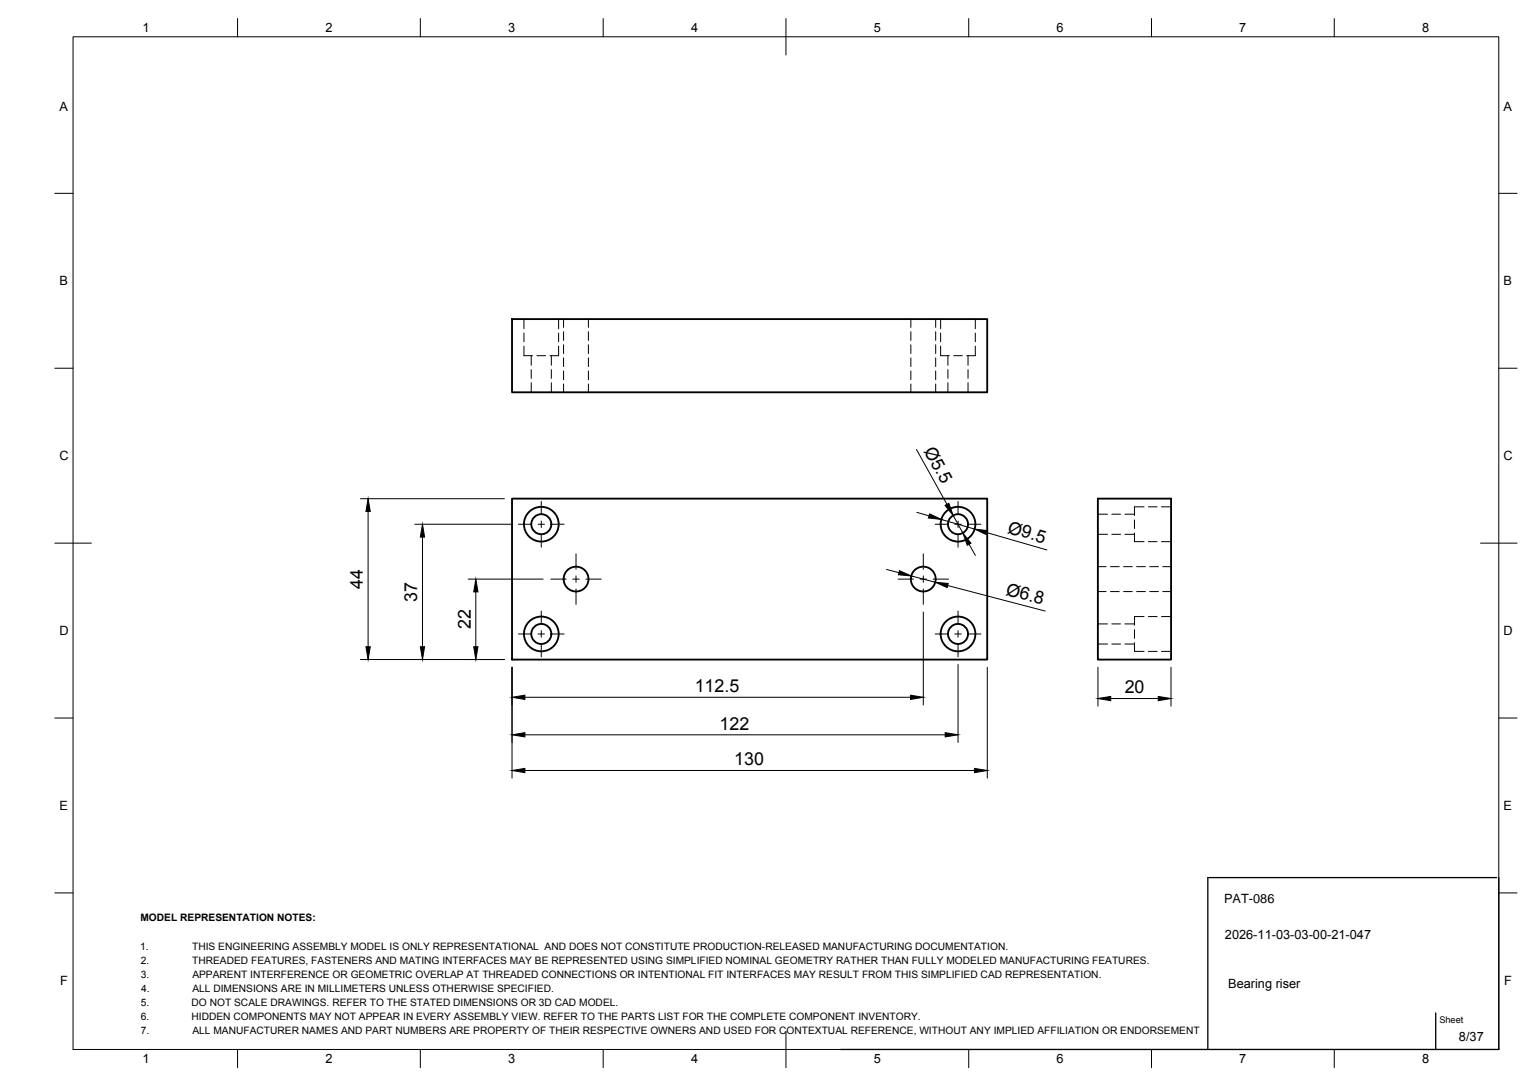
ISO-10303-21;
HEADER;
/* Generated by software containing ST-Developer
 * from STEP Tools, Inc. (www.steptools.com) 
 */

FILE_DESCRIPTION(
/* description */ ('Ratchet and pawl hand winch drum'),
/* implementation_level */ '2;1');

FILE_NAME(
/* name */ 'Bearing riser.step',
/* time_stamp */ '2026-10-27T12:42:58-07:00',
/* author */ (''),
/* organization */ (''),
/* preprocessor_version */ 'ST-DEVELOPER v20.2',
/* originating_system */ 'Autodesk Translation Framework v15.17.0.0',
/* authorisation */ '');

FILE_SCHEMA (('AUTOMOTIVE_DESIGN { 1 0 10303 214 3 1 1 }'));
ENDSEC;

DATA;
#10=MECHANICAL_DESIGN_GEOMETRIC_PRESENTATION_REPRESENTATION('',(#392),#11801);
#324=SHAPE_REPRESENTATION_RELATIONSHIP('SRR','None',#11950,#358);
#358=ADVANCED_BREP_SHAPE_REPRESENTATION('',(#427),#11767);
#392=STYLED_ITEM('',(#12213),#427);
#427=MANIFOLD_SOLID_BREP('Body1',#6269);
#476=FACE_BOUND('',#1246,.T.);
#477=FACE_BOUND('',#1249,.T.);
#478=FACE_BOUND('',#1254,.T.);
#479=FACE_BOUND('',#1257,.T.);
#480=FACE_BOUND('',#1267,.T.);
#481=FACE_BOUND('',#1268,.T.);
#482=FACE_BOUND('',#1269,.T.);
#483=FACE_BOUND('',#1270,.T.);
#484=FACE_BOUND('',#1271,.T.);
#485=FACE_BOUND('',#1272,.T.);
#486=FACE_BOUND('',#1274,.T.);
#487=FACE_BOUND('',#1275,.T.);
#488=FACE_BOUND('',#1276,.T.);
#489=FACE_BOUND('',#1277,.T.);
#490=FACE_BOUND('',#1278,.T.);
#491=FACE_BOUND('',#1279,.T.);
#619=PLANE('',#6736);
#620=PLANE('',#6741);
#621=PLANE('',#6750);
#622=PLANE('',#6755);
#623=PLANE('',#6767);
#624=PLANE('',#6768);
#625=PLANE('',#6769);
#626=PLANE('',#6770);
#627=PLANE('',#6771);
#628=PLANE('',#6772);
#868=FACE_OUTER_BOUND('',#1244,.T.);
#869=FACE_OUTER_BOUND('',#1245,.T.);
#870=FACE_OUTER_BOUND('',#1247,.T.);
#871=FACE_OUTER_BOUND('',#1248,.T.);
#872=FACE_OUTER_BOUND('',#1250,.T.);
#873=FACE_OUTER_BOUND('',#1251,.T.);
#874=FACE_OUTER_BOUND('',#1252,.T.);
#875=FACE_OUTER_BOUND('',#1253,.T.);
#876=FACE_OUTER_BOUND('',#1255,.T.);
#877=FACE_OUTER_BOUND('',#1256,.T.);
#878=FACE_OUTER_BOUND('',#1258,.T.);
#879=FACE_OUTER_BOUND('',#1259,.T.);
#880=FACE_OUTER_BOUND('',#1260,.T.);
#881=FACE_OUTER_BOUND('',#1261,.T.);
#882=FACE_OUTER_BOUND('',#1262,.T.);
#883=FACE_OUTER_BOUND('',#1263,.T.);
#884=FACE_OUTER_BOUND('',#1264,.T.);
#885=FACE_OUTER_BOUND('',#1265,.T.);
#886=FACE_OUTER_BOUND('',#1266,.T.);
#887=FACE_OUTER_BOUND('',#1273,.T.);
#1244=EDGE_LOOP('',(#4379,#4380,#4381,#4382));
#1245=EDGE_LOOP('',(#4383));
#1246=EDGE_LOOP('',(#4384));
#1247=EDGE_LOOP('',(#4385,#4386,#4387,#4388));
#1248=EDGE_LOOP('',(#4389));
#1249=EDGE_LOOP('',(#4390));
#1250=EDGE_LOOP('',(#4391,#4392,#4393,#4394));
#1251=EDGE_LOOP('',(#4395,#4396,#4397,#4398));
#1252=EDGE_LOOP('',(#4399,#4400,#4401,#4402));
#1253=EDGE_LOOP('',(#4403));
#1254=EDGE_LOOP('',(#4404));
#1255=EDGE_LOOP('',(#4405,#4406,#4407,#4408));
#1256=EDGE_LOOP('',(#4409));
#1257=EDGE_LOOP('',(#4410));
#1258=EDGE_LOOP('',(#4411,#4412,#4413,#4414));
#1259=EDGE_LOOP('',(#4415,#4416,#4417,#4418));
#1260=EDGE_LOOP('',(#4419,#4420,#4421,#4422));
#1261=EDGE_LOOP('',(#4423,#4424,#4425,#4426));
#1262=EDGE_LOOP('',(#4427,#4428,#4429,#4430));
#1263=EDGE_LOOP('',(#4431,#4432,#4433,#4434));
#1264=EDGE_LOOP('',(#4435,#4436,#4437,#4438));
#1265=EDGE_LOOP('',(#4439,#4440,#4441,#4442));
#1266=EDGE_LOOP('',(#4443,#4444,#4445,#4446));
#1267=EDGE_LOOP('',(#4447));
#1268=EDGE_LOOP('',(#4448));
#1269=EDGE_LOOP('',(#4449));
#1270=EDGE_LOOP('',(#4450));
#1271=EDGE_LOOP('',(#4451));
#1272=EDGE_LOOP('',(#4452));
#1273=EDGE_LOOP('',(#4453,#4454,#4455,#4456));
#1274=EDGE_LOOP('',(#4457));
#1275=EDGE_LOOP('',(#4458));
#1276=EDGE_LOOP('',(#4459));
#1277=EDGE_LOOP('',(#4460));
#1278=EDGE_LOOP('',(#4461));
#1279=EDGE_LOOP('',(#4462));
#1743=LINE('',#9375,#2254);
#1744=LINE('',#9384,#2255);
#1745=LINE('',#9392,#2256);
#1746=LINE('',#9396,#2257);
#1747=LINE('',#9401,#2258);
#1748=LINE('',#9410,#2259);
#1749=LINE('',#9418,#2260);
#1750=LINE('',#9422,#2261);
#1751=LINE('',#9427,#2262);
#1752=LINE('',#9433,#2263);
#1753=LINE('',#9438,#2264);
#1754=LINE('',#9440,#2265);
#1755=LINE('',#9442,#2266);
#1756=LINE('',#9443,#2267);
#1757=LINE('',#9446,#2268);
#1758=LINE('',#9448,#2269);
#1759=LINE('',#9449,#2270);
#1760=LINE('',#9452,#2271);
#1761=LINE('',#9454,#2272);
#1762=LINE('',#9455,#2273);
#1763=LINE('',#9457,#2274);
#1764=LINE('',#9458,#2275);
#2254=VECTOR('',#7516,0.475);
#2255=VECTOR('',#7527,0.475);
#2256=VECTOR('',#7538,0.275);
#2257=VECTOR('',#7543,0.275);
#2258=VECTOR('',#7548,0.475);
#2259=VECTOR('',#7559,0.475);
#2260=VECTOR('',#7570,0.275);
#2261=VECTOR('',#7575,0.275);
#2262=VECTOR('',#7580,0.34);
#2263=VECTOR('',#7587,0.34);
#2264=VECTOR('',#7592,1.);
#2265=VECTOR('',#7593,1.);
#2266=VECTOR('',#7594,1.);
#2267=VECTOR('',#7595,1.);
#2268=VECTOR('',#7598,1.);
#2269=VECTOR('',#7599,1.);
#2270=VECTOR('',#7600,1.);
#2271=VECTOR('',#7603,1.);
#2272=VECTOR('',#7604,1.);
#2273=VECTOR('',#7605,1.);
#2274=VECTOR('',#7608,1.);
#2275=VECTOR('',#7609,1.);
#2739=CIRCLE('',#6734,0.475);
#2740=CIRCLE('',#6735,0.475);
#2741=CIRCLE('',#6737,0.275);
#2742=CIRCLE('',#6739,0.475);
#2743=CIRCLE('',#6740,0.475);
#2744=CIRCLE('',#6742,0.275);
#2745=CIRCLE('',#6744,0.275);
#2746=CIRCLE('',#6746,0.275);
#2747=CIRCLE('',#6748,0.475);
#2748=CIRCLE('',#6749,0.475);
#2749=CIRCLE('',#6751,0.275);
#2750=CIRCLE('',#6753,0.475);
#2751=CIRCLE('',#6754,0.475);
#2752=CIRCLE('',#6756,0.275);
#2753=CIRCLE('',#6758,0.275);
#2754=CIRCLE('',#6760,0.275);
#2755=CIRCLE('',#6762,0.34);
#2756=CIRCLE('',#6763,0.34);
#2757=CIRCLE('',#6765,0.34);
#2758=CIRCLE('',#6766,0.34);
#2986=VERTEX_POINT('',#9372);
#2987=VERTEX_POINT('',#9374);
#2988=VERTEX_POINT('',#9378);
#2989=VERTEX_POINT('',#9381);
#2990=VERTEX_POINT('',#9383);
#2991=VERTEX_POINT('',#9387);
#2992=VERTEX_POINT('',#9390);
#2993=VERTEX_POINT('',#9394);
#2994=VERTEX_POINT('',#9398);
#2995=VERTEX_POINT('',#9400);
#2996=VERTEX_POINT('',#9404);
#2997=VERTEX_POINT('',#9407);
#2998=VERTEX_POINT('',#9409);
#2999=VERTEX_POINT('',#9413);
#3000=VERTEX_POINT('',#9416);
#3001=VERTEX_POINT('',#9420);
#3002=VERTEX_POINT('',#9424);
#3003=VERTEX_POINT('',#9426);
#3004=VERTEX_POINT('',#9430);
#3005=VERTEX_POINT('',#9432);
#3006=VERTEX_POINT('',#9436);
#3007=VERTEX_POINT('',#9437);
#3008=VERTEX_POINT('',#9439);
#3009=VERTEX_POINT('',#9441);
#3010=VERTEX_POINT('',#9445);
#3011=VERTEX_POINT('',#9447);
#3012=VERTEX_POINT('',#9451);
#3013=VERTEX_POINT('',#9453);
#3533=EDGE_CURVE('',#2986,#2986,#2739,.T.);
#3534=EDGE_CURVE('',#2986,#2987,#1743,.T.);
#3535=EDGE_CURVE('',#2987,#2987,#2740,.T.);
#3536=EDGE_CURVE('',#2988,#2988,#2741,.T.);
#3537=EDGE_CURVE('',#2989,#2989,#2742,.T.);
#3538=EDGE_CURVE('',#2989,#2990,#1744,.T.);
#3539=EDGE_CURVE('',#2990,#2990,#2743,.T.);
#3540=EDGE_CURVE('',#2991,#2991,#2744,.T.);
#3541=EDGE_CURVE('',#2992,#2992,#2745,.T.);
#3542=EDGE_CURVE('',#2992,#2988,#1745,.T.);
#3543=EDGE_CURVE('',#2993,#2993,#2746,.T.);
#3544=EDGE_CURVE('',#2993,#2991,#1746,.T.);
#3545=EDGE_CURVE('',#2994,#2994,#2747,.T.);
#3546=EDGE_CURVE('',#2994,#2995,#1747,.T.);
#3547=EDGE_CURVE('',#2995,#2995,#2748,.T.);
#3548=EDGE_CURVE('',#2996,#2996,#2749,.T.);
#3549=EDGE_CURVE('',#2997,#2997,#2750,.T.);
#3550=EDGE_CURVE('',#2997,#2998,#1748,.T.);
#3551=EDGE_CURVE('',#2998,#2998,#2751,.T.);
#3552=EDGE_CURVE('',#2999,#2999,#2752,.T.);
#3553=EDGE_CURVE('',#3000,#3000,#2753,.T.);
#3554=EDGE_CURVE('',#3000,#2996,#1749,.T.);
#3555=EDGE_CURVE('',#3001,#3001,#2754,.T.);
#3556=EDGE_CURVE('',#3001,#2999,#1750,.T.);
#3557=EDGE_CURVE('',#3002,#3002,#2755,.T.);
#3558=EDGE_CURVE('',#3002,#3003,#1751,.T.);
#3559=EDGE_CURVE('',#3003,#3003,#2756,.T.);
#3560=EDGE_CURVE('',#3004,#3004,#2757,.T.);
#3561=EDGE_CURVE('',#3004,#3005,#1752,.T.);
#3562=EDGE_CURVE('',#3005,#3005,#2758,.T.);
#3563=EDGE_CURVE('',#3006,#3007,#1753,.T.);
#3564=EDGE_CURVE('',#3007,#3008,#1754,.T.);
#3565=EDGE_CURVE('',#3009,#3008,#1755,.T.);
#3566=EDGE_CURVE('',#3006,#3009,#1756,.T.);
#3567=EDGE_CURVE('',#3010,#3006,#1757,.T.);
#3568=EDGE_CURVE('',#3011,#3009,#1758,.T.);
#3569=EDGE_CURVE('',#3010,#3011,#1759,.T.);
#3570=EDGE_CURVE('',#3012,#3010,#1760,.T.);
#3571=EDGE_CURVE('',#3013,#3011,#1761,.T.);
#3572=EDGE_CURVE('',#3012,#3013,#1762,.T.);
#3573=EDGE_CURVE('',#3007,#3012,#1763,.T.);
#3574=EDGE_CURVE('',#3008,#3013,#1764,.T.);
#4379=ORIENTED_EDGE('',*,*,#3533,.F.);
#4380=ORIENTED_EDGE('',*,*,#3534,.T.);
#4381=ORIENTED_EDGE('',*,*,#3535,.F.);
#4382=ORIENTED_EDGE('',*,*,#3534,.F.);
#4383=ORIENTED_EDGE('',*,*,#3533,.T.);
#4384=ORIENTED_EDGE('',*,*,#3536,.F.);
#4385=ORIENTED_EDGE('',*,*,#3537,.F.);
#4386=ORIENTED_EDGE('',*,*,#3538,.T.);
#4387=ORIENTED_EDGE('',*,*,#3539,.F.);
#4388=ORIENTED_EDGE('',*,*,#3538,.F.);
#4389=ORIENTED_EDGE('',*,*,#3537,.T.);
#4390=ORIENTED_EDGE('',*,*,#3540,.F.);
#4391=ORIENTED_EDGE('',*,*,#3541,.F.);
#4392=ORIENTED_EDGE('',*,*,#3542,.T.);
#4393=ORIENTED_EDGE('',*,*,#3536,.T.);
#4394=ORIENTED_EDGE('',*,*,#3542,.F.);
#4395=ORIENTED_EDGE('',*,*,#3543,.F.);
#4396=ORIENTED_EDGE('',*,*,#3544,.T.);
#4397=ORIENTED_EDGE('',*,*,#3540,.T.);
#4398=ORIENTED_EDGE('',*,*,#3544,.F.);
#4399=ORIENTED_EDGE('',*,*,#3545,.F.);
#4400=ORIENTED_EDGE('',*,*,#3546,.T.);
#4401=ORIENTED_EDGE('',*,*,#3547,.F.);
#4402=ORIENTED_EDGE('',*,*,#3546,.F.);
#4403=ORIENTED_EDGE('',*,*,#3545,.T.);
#4404=ORIENTED_EDGE('',*,*,#3548,.F.);
#4405=ORIENTED_EDGE('',*,*,#3549,.F.);
#4406=ORIENTED_EDGE('',*,*,#3550,.T.);
#4407=ORIENTED_EDGE('',*,*,#3551,.F.);
#4408=ORIENTED_EDGE('',*,*,#3550,.F.);
#4409=ORIENTED_EDGE('',*,*,#3549,.T.);
#4410=ORIENTED_EDGE('',*,*,#3552,.F.);
#4411=ORIENTED_EDGE('',*,*,#3553,.F.);
#4412=ORIENTED_EDGE('',*,*,#3554,.T.);
#4413=ORIENTED_EDGE('',*,*,#3548,.T.);
#4414=ORIENTED_EDGE('',*,*,#3554,.F.);
#4415=ORIENTED_EDGE('',*,*,#3555,.F.);
#4416=ORIENTED_EDGE('',*,*,#3556,.T.);
#4417=ORIENTED_EDGE('',*,*,#3552,.T.);
#4418=ORIENTED_EDGE('',*,*,#3556,.F.);
#4419=ORIENTED_EDGE('',*,*,#3557,.F.);
#4420=ORIENTED_EDGE('',*,*,#3558,.T.);
#4421=ORIENTED_EDGE('',*,*,#3559,.F.);
#4422=ORIENTED_EDGE('',*,*,#3558,.F.);
#4423=ORIENTED_EDGE('',*,*,#3560,.F.);
#4424=ORIENTED_EDGE('',*,*,#3561,.T.);
#4425=ORIENTED_EDGE('',*,*,#3562,.F.);
#4426=ORIENTED_EDGE('',*,*,#3561,.F.);
#4427=ORIENTED_EDGE('',*,*,#3563,.T.);
#4428=ORIENTED_EDGE('',*,*,#3564,.T.);
#4429=ORIENTED_EDGE('',*,*,#3565,.F.);
#4430=ORIENTED_EDGE('',*,*,#3566,.F.);
#4431=ORIENTED_EDGE('',*,*,#3567,.T.);
#4432=ORIENTED_EDGE('',*,*,#3566,.T.);
#4433=ORIENTED_EDGE('',*,*,#3568,.F.);
#4434=ORIENTED_EDGE('',*,*,#3569,.F.);
#4435=ORIENTED_EDGE('',*,*,#3570,.T.);
#4436=ORIENTED_EDGE('',*,*,#3569,.T.);
#4437=ORIENTED_EDGE('',*,*,#3571,.F.);
#4438=ORIENTED_EDGE('',*,*,#3572,.F.);
#4439=ORIENTED_EDGE('',*,*,#3573,.T.);
#4440=ORIENTED_EDGE('',*,*,#3572,.T.);
#4441=ORIENTED_EDGE('',*,*,#3574,.F.);
#4442=ORIENTED_EDGE('',*,*,#3564,.F.);
#4443=ORIENTED_EDGE('',*,*,#3574,.T.);
#4444=ORIENTED_EDGE('',*,*,#3571,.T.);
#4445=ORIENTED_EDGE('',*,*,#3568,.T.);
#4446=ORIENTED_EDGE('',*,*,#3565,.T.);
#4447=ORIENTED_EDGE('',*,*,#3562,.T.);
#4448=ORIENTED_EDGE('',*,*,#3559,.T.);
#4449=ORIENTED_EDGE('',*,*,#3551,.T.);
#4450=ORIENTED_EDGE('',*,*,#3547,.T.);
#4451=ORIENTED_EDGE('',*,*,#3539,.T.);
#4452=ORIENTED_EDGE('',*,*,#3535,.T.);
#4453=ORIENTED_EDGE('',*,*,#3573,.F.);
#4454=ORIENTED_EDGE('',*,*,#3563,.F.);
#4455=ORIENTED_EDGE('',*,*,#3567,.F.);
#4456=ORIENTED_EDGE('',*,*,#3570,.F.);
#4457=ORIENTED_EDGE('',*,*,#3541,.T.);
#4458=ORIENTED_EDGE('',*,*,#3543,.T.);
#4459=ORIENTED_EDGE('',*,*,#3553,.T.);
#4460=ORIENTED_EDGE('',*,*,#3555,.T.);
#4461=ORIENTED_EDGE('',*,*,#3557,.T.);
#4462=ORIENTED_EDGE('',*,*,#3560,.T.);
#5817=CYLINDRICAL_SURFACE('',#6733,0.475);
#5818=CYLINDRICAL_SURFACE('',#6738,0.475);
#5819=CYLINDRICAL_SURFACE('',#6743,0.275);
#5820=CYLINDRICAL_SURFACE('',#6745,0.275);
#5821=CYLINDRICAL_SURFACE('',#6747,0.475);
#5822=CYLINDRICAL_SURFACE('',#6752,0.475);
#5823=CYLINDRICAL_SURFACE('',#6757,0.275);
#5824=CYLINDRICAL_SURFACE('',#6759,0.275);
#5825=CYLINDRICAL_SURFACE('',#6761,0.34);
#5826=CYLINDRICAL_SURFACE('',#6764,0.34);
#5938=ADVANCED_FACE('',(#868),#5817,.F.);
#5939=ADVANCED_FACE('',(#869,#476),#619,.T.);
#5940=ADVANCED_FACE('',(#870),#5818,.F.);
#5941=ADVANCED_FACE('',(#871,#477),#620,.T.);
#5942=ADVANCED_FACE('',(#872),#5819,.F.);
#5943=ADVANCED_FACE('',(#873),#5820,.F.);
#5944=ADVANCED_FACE('',(#874),#5821,.F.);
#5945=ADVANCED_FACE('',(#875,#478),#621,.T.);
#5946=ADVANCED_FACE('',(#876),#5822,.F.);
#5947=ADVANCED_FACE('',(#877,#479),#622,.T.);
#5948=ADVANCED_FACE('',(#878),#5823,.F.);
#5949=ADVANCED_FACE('',(#879),#5824,.F.);
#5950=ADVANCED_FACE('',(#880),#5825,.F.);
#5951=ADVANCED_FACE('',(#881),#5826,.F.);
#5952=ADVANCED_FACE('',(#882),#623,.T.);
#5953=ADVANCED_FACE('',(#883),#624,.T.);
#5954=ADVANCED_FACE('',(#884),#625,.T.);
#5955=ADVANCED_FACE('',(#885),#626,.T.);
#5956=ADVANCED_FACE('',(#886,#480,#481,#482,#483,#484,#485),#627,.T.);
#5957=ADVANCED_FACE('',(#887,#486,#487,#488,#489,#490,#491),#628,.F.);
#6269=CLOSED_SHELL('',(#5938,#5939,#5940,#5941,#5942,#5943,#5944,#5945,
#5946,#5947,#5948,#5949,#5950,#5951,#5952,#5953,#5954,#5955,#5956,#5957));
#6732=AXIS2_PLACEMENT_3D('',#9370,#7510,#7511);
#6733=AXIS2_PLACEMENT_3D('',#9371,#7512,#7513);
#6734=AXIS2_PLACEMENT_3D('',#9373,#7514,#7515);
#6735=AXIS2_PLACEMENT_3D('',#9376,#7517,#7518);
#6736=AXIS2_PLACEMENT_3D('',#9377,#7519,#7520);
#6737=AXIS2_PLACEMENT_3D('',#9379,#7521,#7522);
#6738=AXIS2_PLACEMENT_3D('',#9380,#7523,#7524);
#6739=AXIS2_PLACEMENT_3D('',#9382,#7525,#7526);
#6740=AXIS2_PLACEMENT_3D('',#9385,#7528,#7529);
#6741=AXIS2_PLACEMENT_3D('',#9386,#7530,#7531);
#6742=AXIS2_PLACEMENT_3D('',#9388,#7532,#7533);
#6743=AXIS2_PLACEMENT_3D('',#9389,#7534,#7535);
#6744=AXIS2_PLACEMENT_3D('',#9391,#7536,#7537);
#6745=AXIS2_PLACEMENT_3D('',#9393,#7539,#7540);
#6746=AXIS2_PLACEMENT_3D('',#9395,#7541,#7542);
#6747=AXIS2_PLACEMENT_3D('',#9397,#7544,#7545);
#6748=AXIS2_PLACEMENT_3D('',#9399,#7546,#7547);
#6749=AXIS2_PLACEMENT_3D('',#9402,#7549,#7550);
#6750=AXIS2_PLACEMENT_3D('',#9403,#7551,#7552);
#6751=AXIS2_PLACEMENT_3D('',#9405,#7553,#7554);
#6752=AXIS2_PLACEMENT_3D('',#9406,#7555,#7556);
#6753=AXIS2_PLACEMENT_3D('',#9408,#7557,#7558);
#6754=AXIS2_PLACEMENT_3D('',#9411,#7560,#7561);
#6755=AXIS2_PLACEMENT_3D('',#9412,#7562,#7563);
#6756=AXIS2_PLACEMENT_3D('',#9414,#7564,#7565);
#6757=AXIS2_PLACEMENT_3D('',#9415,#7566,#7567);
#6758=AXIS2_PLACEMENT_3D('',#9417,#7568,#7569);
#6759=AXIS2_PLACEMENT_3D('',#9419,#7571,#7572);
#6760=AXIS2_PLACEMENT_3D('',#9421,#7573,#7574);
#6761=AXIS2_PLACEMENT_3D('',#9423,#7576,#7577);
#6762=AXIS2_PLACEMENT_3D('',#9425,#7578,#7579);
#6763=AXIS2_PLACEMENT_3D('',#9428,#7581,#7582);
#6764=AXIS2_PLACEMENT_3D('',#9429,#7583,#7584);
#6765=AXIS2_PLACEMENT_3D('',#9431,#7585,#7586);
#6766=AXIS2_PLACEMENT_3D('',#9434,#7588,#7589);
#6767=AXIS2_PLACEMENT_3D('',#9435,#7590,#7591);
#6768=AXIS2_PLACEMENT_3D('',#9444,#7596,#7597);
#6769=AXIS2_PLACEMENT_3D('',#9450,#7601,#7602);
#6770=AXIS2_PLACEMENT_3D('',#9456,#7606,#7607);
#6771=AXIS2_PLACEMENT_3D('',#9459,#7610,#7611);
#6772=AXIS2_PLACEMENT_3D('',#9460,#7612,#7613);
#7510=DIRECTION('axis',(0.,0.,1.));
#7511=DIRECTION('refdir',(1.,0.,0.));
#7512=DIRECTION('center_axis',(0.,0.,1.));
#7513=DIRECTION('ref_axis',(1.,0.,0.));
#7514=DIRECTION('center_axis',(0.,0.,1.));
#7515=DIRECTION('ref_axis',(1.,0.,0.));
#7516=DIRECTION('',(0.,0.,1.));
#7517=DIRECTION('center_axis',(0.,0.,-1.));
#7518=DIRECTION('ref_axis',(1.,0.,0.));
#7519=DIRECTION('center_axis',(0.,0.,1.));
#7520=DIRECTION('ref_axis',(1.,0.,0.));
#7521=DIRECTION('center_axis',(0.,0.,1.));
#7522=DIRECTION('ref_axis',(1.,0.,0.));
#7523=DIRECTION('center_axis',(0.,0.,1.));
#7524=DIRECTION('ref_axis',(1.,0.,0.));
#7525=DIRECTION('center_axis',(0.,0.,1.));
#7526=DIRECTION('ref_axis',(1.,0.,0.));
#7527=DIRECTION('',(0.,0.,1.));
#7528=DIRECTION('center_axis',(0.,0.,-1.));
#7529=DIRECTION('ref_axis',(1.,0.,0.));
#7530=DIRECTION('center_axis',(0.,0.,1.));
#7531=DIRECTION('ref_axis',(1.,0.,0.));
#7532=DIRECTION('center_axis',(0.,0.,1.));
#7533=DIRECTION('ref_axis',(1.,0.,0.));
#7534=DIRECTION('center_axis',(0.,0.,1.));
#7535=DIRECTION('ref_axis',(1.,0.,0.));
#7536=DIRECTION('center_axis',(0.,0.,1.));
#7537=DIRECTION('ref_axis',(1.,0.,0.));
#7538=DIRECTION('',(0.,0.,1.));
#7539=DIRECTION('center_axis',(0.,0.,1.));
#7540=DIRECTION('ref_axis',(1.,0.,0.));
#7541=DIRECTION('center_axis',(0.,0.,1.));
#7542=DIRECTION('ref_axis',(1.,0.,0.));
#7543=DIRECTION('',(0.,0.,1.));
#7544=DIRECTION('center_axis',(0.,0.,1.));
#7545=DIRECTION('ref_axis',(1.,0.,0.));
#7546=DIRECTION('center_axis',(0.,0.,1.));
#7547=DIRECTION('ref_axis',(1.,0.,0.));
#7548=DIRECTION('',(0.,0.,1.));
#7549=DIRECTION('center_axis',(0.,0.,-1.));
#7550=DIRECTION('ref_axis',(1.,0.,0.));
#7551=DIRECTION('center_axis',(0.,0.,1.));
#7552=DIRECTION('ref_axis',(1.,0.,0.));
#7553=DIRECTION('center_axis',(0.,0.,1.));
#7554=DIRECTION('ref_axis',(1.,0.,0.));
#7555=DIRECTION('center_axis',(0.,0.,1.));
#7556=DIRECTION('ref_axis',(1.,0.,0.));
#7557=DIRECTION('center_axis',(0.,0.,1.));
#7558=DIRECTION('ref_axis',(1.,0.,0.));
#7559=DIRECTION('',(0.,0.,1.));
#7560=DIRECTION('center_axis',(0.,0.,-1.));
#7561=DIRECTION('ref_axis',(1.,0.,0.));
#7562=DIRECTION('center_axis',(0.,0.,1.));
#7563=DIRECTION('ref_axis',(1.,0.,0.));
#7564=DIRECTION('center_axis',(0.,0.,1.));
#7565=DIRECTION('ref_axis',(1.,0.,0.));
#7566=DIRECTION('center_axis',(0.,0.,1.));
#7567=DIRECTION('ref_axis',(1.,0.,0.));
#7568=DIRECTION('center_axis',(0.,0.,1.));
#7569=DIRECTION('ref_axis',(1.,0.,0.));
#7570=DIRECTION('',(0.,0.,1.));
#7571=DIRECTION('center_axis',(0.,0.,1.));
#7572=DIRECTION('ref_axis',(1.,0.,0.));
#7573=DIRECTION('center_axis',(0.,0.,1.));
#7574=DIRECTION('ref_axis',(1.,0.,0.));
#7575=DIRECTION('',(0.,0.,1.));
#7576=DIRECTION('center_axis',(0.,0.,1.));
#7577=DIRECTION('ref_axis',(1.,0.,0.));
#7578=DIRECTION('center_axis',(0.,0.,1.));
#7579=DIRECTION('ref_axis',(1.,0.,0.));
#7580=DIRECTION('',(0.,0.,1.));
#7581=DIRECTION('center_axis',(0.,0.,-1.));
#7582=DIRECTION('ref_axis',(1.,0.,0.));
#7583=DIRECTION('center_axis',(0.,0.,1.));
#7584=DIRECTION('ref_axis',(1.,0.,0.));
#7585=DIRECTION('center_axis',(0.,0.,1.));
#7586=DIRECTION('ref_axis',(1.,0.,0.));
#7587=DIRECTION('',(0.,0.,1.));
#7588=DIRECTION('center_axis',(0.,0.,-1.));
#7589=DIRECTION('ref_axis',(1.,0.,0.));
#7590=DIRECTION('center_axis',(0.,1.,0.));
#7591=DIRECTION('ref_axis',(-1.,0.,0.));
#7592=DIRECTION('',(-1.,0.,0.));
#7593=DIRECTION('',(0.,0.,1.));
#7594=DIRECTION('',(-1.,0.,0.));
#7595=DIRECTION('',(0.,0.,1.));
#7596=DIRECTION('center_axis',(1.,0.,0.));
#7597=DIRECTION('ref_axis',(0.,1.,0.));
#7598=DIRECTION('',(0.,1.,0.));
#7599=DIRECTION('',(0.,1.,0.));
#7600=DIRECTION('',(0.,0.,1.));
#7601=DIRECTION('center_axis',(0.,-1.,0.));
#7602=DIRECTION('ref_axis',(1.,0.,0.));
#7603=DIRECTION('',(1.,0.,0.));
#7604=DIRECTION('',(1.,0.,0.));
#7605=DIRECTION('',(0.,0.,1.));
#7606=DIRECTION('center_axis',(-1.,0.,0.));
#7607=DIRECTION('ref_axis',(0.,-1.,0.));
#7608=DIRECTION('',(0.,-1.,0.));
#7609=DIRECTION('',(0.,-1.,0.));
#7610=DIRECTION('center_axis',(0.,0.,1.));
#7611=DIRECTION('ref_axis',(1.,0.,0.));
#7612=DIRECTION('center_axis',(0.,0.,1.));
#7613=DIRECTION('ref_axis',(1.,0.,0.));
#9370=CARTESIAN_POINT('',(0.,0.,0.));
#9371=CARTESIAN_POINT('Origin',(5.7,-1.5,2.2));
#9372=CARTESIAN_POINT('',(5.225,-1.5,2.2));
#9373=CARTESIAN_POINT('Origin',(5.7,-1.5,2.2));
#9374=CARTESIAN_POINT('',(5.225,-1.5,3.2));
#9375=CARTESIAN_POINT('',(5.225,-1.5,2.2));
#9376=CARTESIAN_POINT('Origin',(5.7,-1.5,3.2));
#9377=CARTESIAN_POINT('Origin',(5.7,-1.5,2.2));
#9378=CARTESIAN_POINT('',(5.425,-1.5,2.2));
#9379=CARTESIAN_POINT('Origin',(5.7,-1.5,2.2));
#9380=CARTESIAN_POINT('Origin',(5.7,1.5,2.2));
#9381=CARTESIAN_POINT('',(5.225,1.5,2.2));
#9382=CARTESIAN_POINT('Origin',(5.7,1.5,2.2));
#9383=CARTESIAN_POINT('',(5.225,1.5,3.2));
#9384=CARTESIAN_POINT('',(5.225,1.5,2.2));
#9385=CARTESIAN_POINT('Origin',(5.7,1.5,3.2));
#9386=CARTESIAN_POINT('Origin',(5.7,1.5,2.2));
#9387=CARTESIAN_POINT('',(5.425,1.5,2.2));
#9388=CARTESIAN_POINT('Origin',(5.7,1.5,2.2));
#9389=CARTESIAN_POINT('Origin',(5.7,-1.5,1.1));
#9390=CARTESIAN_POINT('',(5.425,-1.5,1.2));
#9391=CARTESIAN_POINT('Origin',(5.7,-1.5,1.2));
#9392=CARTESIAN_POINT('',(5.425,-1.5,1.1));
#9393=CARTESIAN_POINT('Origin',(5.7,1.5,1.1));
#9394=CARTESIAN_POINT('',(5.425,1.5,1.2));
#9395=CARTESIAN_POINT('Origin',(5.7,1.5,1.2));
#9396=CARTESIAN_POINT('',(5.425,1.5,1.1));
#9397=CARTESIAN_POINT('Origin',(-5.7,-1.5,2.2));
#9398=CARTESIAN_POINT('',(-6.175,-1.5,2.2));
#9399=CARTESIAN_POINT('Origin',(-5.7,-1.5,2.2));
#9400=CARTESIAN_POINT('',(-6.175,-1.5,3.2));
#9401=CARTESIAN_POINT('',(-6.175,-1.5,2.2));
#9402=CARTESIAN_POINT('Origin',(-5.7,-1.5,3.2));
#9403=CARTESIAN_POINT('Origin',(-5.7,-1.5,2.2));
#9404=CARTESIAN_POINT('',(-5.975,-1.5,2.2));
#9405=CARTESIAN_POINT('Origin',(-5.7,-1.5,2.2));
#9406=CARTESIAN_POINT('Origin',(-5.7,1.5,2.2));
#9407=CARTESIAN_POINT('',(-6.175,1.5,2.2));
#9408=CARTESIAN_POINT('Origin',(-5.7,1.5,2.2));
#9409=CARTESIAN_POINT('',(-6.175,1.5,3.2));
#9410=CARTESIAN_POINT('',(-6.175,1.5,2.2));
#9411=CARTESIAN_POINT('Origin',(-5.7,1.5,3.2));
#9412=CARTESIAN_POINT('Origin',(-5.7,1.5,2.2));
#9413=CARTESIAN_POINT('',(-5.975,1.5,2.2));
#9414=CARTESIAN_POINT('Origin',(-5.7,1.5,2.2));
#9415=CARTESIAN_POINT('Origin',(-5.7,-1.5,1.1));
#9416=CARTESIAN_POINT('',(-5.975,-1.5,1.2));
#9417=CARTESIAN_POINT('Origin',(-5.7,-1.5,1.2));
#9418=CARTESIAN_POINT('',(-5.975,-1.5,1.1));
#9419=CARTESIAN_POINT('Origin',(-5.7,1.5,1.1));
#9420=CARTESIAN_POINT('',(-5.975,1.5,1.2));
#9421=CARTESIAN_POINT('Origin',(-5.7,1.5,1.2));
#9422=CARTESIAN_POINT('',(-5.975,1.5,1.1));
#9423=CARTESIAN_POINT('Origin',(-4.75,0.,1.1));
#9424=CARTESIAN_POINT('',(-5.09,-4.163799117101E-17,1.2));
#9425=CARTESIAN_POINT('Origin',(-4.75,0.,1.2));
#9426=CARTESIAN_POINT('',(-5.09,4.163799117101E-17,3.2));
#9427=CARTESIAN_POINT('',(-5.09,-4.163799117101E-17,1.1));
#9428=CARTESIAN_POINT('Origin',(-4.75,0.,3.2));
#9429=CARTESIAN_POINT('Origin',(4.75,0.,1.1));
#9430=CARTESIAN_POINT('',(4.41,-4.163799117101E-17,1.2));
#9431=CARTESIAN_POINT('Origin',(4.75,0.,1.2));
#9432=CARTESIAN_POINT('',(4.41,4.163799117101E-17,3.2));
#9433=CARTESIAN_POINT('',(4.41,-4.163799117101E-17,1.1));
#9434=CARTESIAN_POINT('Origin',(4.75,0.,3.2));
#9435=CARTESIAN_POINT('Origin',(6.5,2.2,1.2));
#9436=CARTESIAN_POINT('',(6.5,2.2,1.2));
#9437=CARTESIAN_POINT('',(-6.5,2.2,1.2));
#9438=CARTESIAN_POINT('',(6.5,2.2,1.2));
#9439=CARTESIAN_POINT('',(-6.5,2.2,3.2));
#9440=CARTESIAN_POINT('',(-6.5,2.2,1.2));
#9441=CARTESIAN_POINT('',(6.5,2.2,3.2));
#9442=CARTESIAN_POINT('',(6.5,2.2,3.2));
#9443=CARTESIAN_POINT('',(6.5,2.2,1.2));
#9444=CARTESIAN_POINT('Origin',(6.5,-2.2,1.2));
#9445=CARTESIAN_POINT('',(6.5,-2.2,1.2));
#9446=CARTESIAN_POINT('',(6.5,-2.2,1.2));
#9447=CARTESIAN_POINT('',(6.5,-2.2,3.2));
#9448=CARTESIAN_POINT('',(6.5,-2.2,3.2));
#9449=CARTESIAN_POINT('',(6.5,-2.2,1.2));
#9450=CARTESIAN_POINT('Origin',(-6.5,-2.2,1.2));
#9451=CARTESIAN_POINT('',(-6.5,-2.2,1.2));
#9452=CARTESIAN_POINT('',(-6.5,-2.2,1.2));
#9453=CARTESIAN_POINT('',(-6.5,-2.2,3.2));
#9454=CARTESIAN_POINT('',(-6.5,-2.2,3.2));
#9455=CARTESIAN_POINT('',(-6.5,-2.2,1.2));
#9456=CARTESIAN_POINT('Origin',(-6.5,2.2,1.2));
#9457=CARTESIAN_POINT('',(-6.5,2.2,1.2));
#9458=CARTESIAN_POINT('',(-6.5,2.2,3.2));
#9459=CARTESIAN_POINT('Origin',(0.,0.,3.2));
#9460=CARTESIAN_POINT('Origin',(0.,0.,1.2));
#11727=UNCERTAINTY_MEASURE_WITH_UNIT(LENGTH_MEASURE(0.001),#11802,
'DISTANCE_ACCURACY_VALUE',
'Maximum model space distance between geometric entities at asserted c
onnectivities');
#11761=UNCERTAINTY_MEASURE_WITH_UNIT(LENGTH_MEASURE(0.001),#11802,
'DISTANCE_ACCURACY_VALUE',
'Maximum model space distance between geometric entities at asserted c
onnectivities');
#11767=(
GEOMETRIC_REPRESENTATION_CONTEXT(3)
GLOBAL_UNCERTAINTY_ASSIGNED_CONTEXT((#11727))
GLOBAL_UNIT_ASSIGNED_CONTEXT((#11802,#11804,#11805))
REPRESENTATION_CONTEXT('','3D')
);
#11801=(
GEOMETRIC_REPRESENTATION_CONTEXT(3)
GLOBAL_UNCERTAINTY_ASSIGNED_CONTEXT((#11761))
GLOBAL_UNIT_ASSIGNED_CONTEXT((#11802,#11804,#11805))
REPRESENTATION_CONTEXT('','3D')
);
#11802=(
LENGTH_UNIT()
NAMED_UNIT(*)
SI_UNIT(.CENTI.,.METRE.)
);
#11804=(
NAMED_UNIT(*)
PLANE_ANGLE_UNIT()
SI_UNIT($,.RADIAN.)
);
#11805=(
NAMED_UNIT(*)
SI_UNIT($,.STERADIAN.)
SOLID_ANGLE_UNIT()
);
#11811=SHAPE_DEFINITION_REPRESENTATION(#11850,#11950);
#11850=PRODUCT_DEFINITION_SHAPE('',$,#11990);
#11950=SHAPE_REPRESENTATION('',(#6732),#11767);
#11984=PRODUCT_DEFINITION_CONTEXT('part definition',#12103,'design');
#11990=PRODUCT_DEFINITION('Bearing riser','Bearing riser',#12029,#11984);
#12029=PRODUCT_DEFINITION_FORMATION('',$,#12110);
#12103=APPLICATION_CONTEXT(
'Core Data for Automotive Mechanical Design Process');
#12104=PRODUCT_CONTEXT('part definition',#12103,'mechanical');
#12110=PRODUCT('Bearing riser','Bearing riser','Bearing riser',(#12104));
#12207=COLOUR_RGB('Grey',0.48,0.52,0.57);
#12208=FILL_AREA_STYLE_COLOUR('',#12207);
#12209=FILL_AREA_STYLE('',(#12208));
#12210=SURFACE_STYLE_FILL_AREA(#12209);
#12211=SURFACE_SIDE_STYLE('',(#12210));
#12212=SURFACE_STYLE_USAGE(.BOTH.,#12211);
#12213=PRESENTATION_STYLE_ASSIGNMENT((#12212));
ENDSEC;
END-ISO-10303-21;
